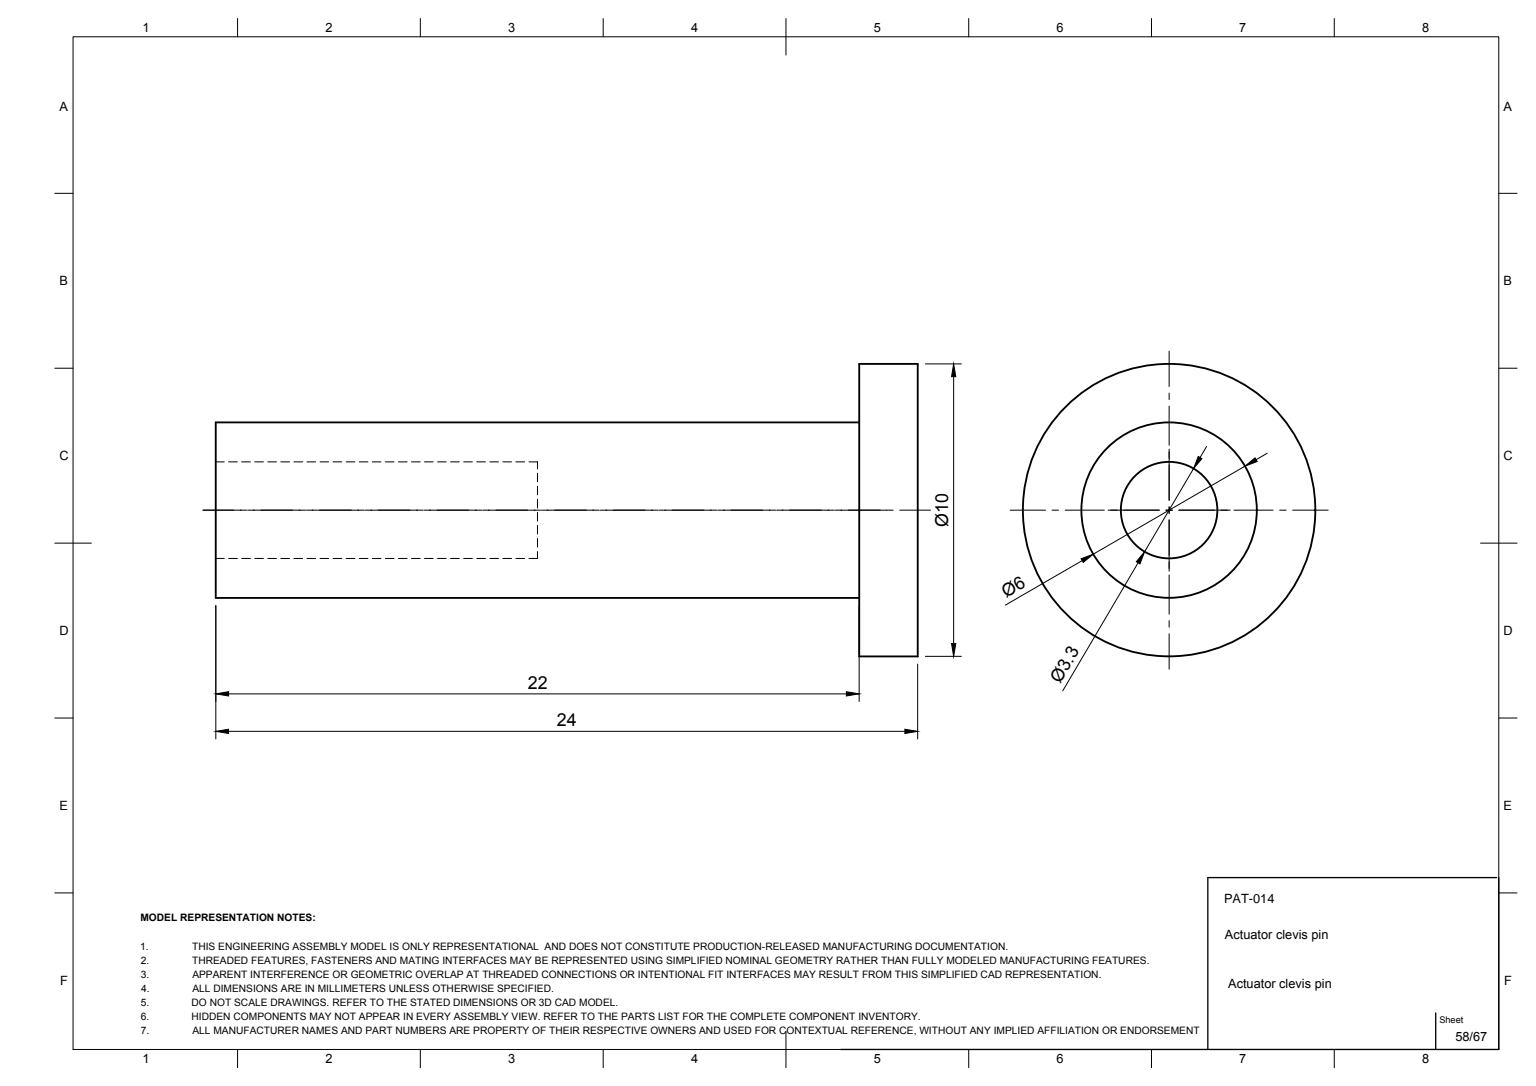
ISO-10303-21;
HEADER;
/* Generated by software containing ST-Developer
 * from STEP Tools, Inc. (www.steptools.com) 
 */

FILE_DESCRIPTION(
/* description */ ('Bin tilter linkage'),
/* implementation_level */ '2;1');

FILE_NAME(
/* name */ 'Actuator clevis pin.step',
/* time_stamp */ '2026-10-28T03:26:24-07:00',
/* author */ (''),
/* organization */ (''),
/* preprocessor_version */ 'ST-DEVELOPER v20.2',
/* originating_system */ 'Autodesk Translation Framework v15.17.0.0',
/* authorisation */ '');

FILE_SCHEMA (('AUTOMOTIVE_DESIGN { 1 0 10303 214 3 1 1 }'));
ENDSEC;

DATA;
#10=MECHANICAL_DESIGN_GEOMETRIC_PRESENTATION_REPRESENTATION('',(#964),#23728);
#744=SHAPE_REPRESENTATION_RELATIONSHIP('SRR','None',#24213,#850);
#850=ADVANCED_BREP_SHAPE_REPRESENTATION('',(#1076),#23713);
#964=STYLED_ITEM('',(#24765),#1076);
#1076=MANIFOLD_SOLID_BREP('Body1',#12496);
#1464=FACE_BOUND('',#3742,.T.);
#1465=FACE_BOUND('',#3747,.T.);
#1840=PLANE('',#15289);
#1841=PLANE('',#15290);
#1842=PLANE('',#15295);
#1843=PLANE('',#15298);
#2585=FACE_OUTER_BOUND('',#3739,.T.);
#2586=FACE_OUTER_BOUND('',#3740,.T.);
#2587=FACE_OUTER_BOUND('',#3741,.T.);
#2588=FACE_OUTER_BOUND('',#3743,.T.);
#2589=FACE_OUTER_BOUND('',#3744,.T.);
#2590=FACE_OUTER_BOUND('',#3745,.T.);
#2591=FACE_OUTER_BOUND('',#3746,.T.);
#3739=EDGE_LOOP('',(#10985,#10986,#10987,#10988));
#3740=EDGE_LOOP('',(#10989));
#3741=EDGE_LOOP('',(#10990));
#3742=EDGE_LOOP('',(#10991));
#3743=EDGE_LOOP('',(#10992,#10993,#10994,#10995));
#3744=EDGE_LOOP('',(#10996));
#3745=EDGE_LOOP('',(#10997,#10998,#10999,#11000));
#3746=EDGE_LOOP('',(#11001));
#3747=EDGE_LOOP('',(#11002));
#4450=LINE('',#23144,#5125);
#4451=LINE('',#23154,#5126);
#4452=LINE('',#23160,#5127);
#5125=VECTOR('',#19299,0.165);
#5126=VECTOR('',#19312,0.5);
#5127=VECTOR('',#19321,0.3);
#5890=CIRCLE('',#15287,0.165);
#5891=CIRCLE('',#15288,0.165);
#5892=CIRCLE('',#15291,0.5);
#5893=CIRCLE('',#15292,0.3);
#5894=CIRCLE('',#15294,0.5);
#5895=CIRCLE('',#15297,0.3);
#6833=VERTEX_POINT('',#23141);
#6834=VERTEX_POINT('',#23143);
#6835=VERTEX_POINT('',#23148);
#6836=VERTEX_POINT('',#23150);
#6837=VERTEX_POINT('',#23153);
#6838=VERTEX_POINT('',#23158);
#8232=EDGE_CURVE('',#6833,#6833,#5890,.T.);
#8233=EDGE_CURVE('',#6833,#6834,#4450,.T.);
#8234=EDGE_CURVE('',#6834,#6834,#5891,.T.);
#8235=EDGE_CURVE('',#6835,#6835,#5892,.T.);
#8236=EDGE_CURVE('',#6836,#6836,#5893,.T.);
#8237=EDGE_CURVE('',#6835,#6837,#4451,.T.);
#8238=EDGE_CURVE('',#6837,#6837,#5894,.T.);
#8239=EDGE_CURVE('',#6838,#6838,#5895,.T.);
#8240=EDGE_CURVE('',#6838,#6836,#4452,.T.);
#10985=ORIENTED_EDGE('',*,*,#8232,.F.);
#10986=ORIENTED_EDGE('',*,*,#8233,.T.);
#10987=ORIENTED_EDGE('',*,*,#8234,.F.);
#10988=ORIENTED_EDGE('',*,*,#8233,.F.);
#10989=ORIENTED_EDGE('',*,*,#8232,.T.);
#10990=ORIENTED_EDGE('',*,*,#8235,.T.);
#10991=ORIENTED_EDGE('',*,*,#8236,.F.);
#10992=ORIENTED_EDGE('',*,*,#8235,.F.);
#10993=ORIENTED_EDGE('',*,*,#8237,.T.);
#10994=ORIENTED_EDGE('',*,*,#8238,.T.);
#10995=ORIENTED_EDGE('',*,*,#8237,.F.);
#10996=ORIENTED_EDGE('',*,*,#8238,.F.);
#10997=ORIENTED_EDGE('',*,*,#8239,.F.);
#10998=ORIENTED_EDGE('',*,*,#8240,.T.);
#10999=ORIENTED_EDGE('',*,*,#8236,.T.);
#11000=ORIENTED_EDGE('',*,*,#8240,.F.);
#11001=ORIENTED_EDGE('',*,*,#8239,.T.);
#11002=ORIENTED_EDGE('',*,*,#8234,.T.);
#11586=CYLINDRICAL_SURFACE('',#15286,0.165);
#11587=CYLINDRICAL_SURFACE('',#15293,0.5);
#11588=CYLINDRICAL_SURFACE('',#15296,0.3);
#12310=ADVANCED_FACE('',(#2585),#11586,.F.);
#12311=ADVANCED_FACE('',(#2586),#1840,.T.);
#12312=ADVANCED_FACE('',(#2587,#1464),#1841,.T.);
#12313=ADVANCED_FACE('',(#2588),#11587,.T.);
#12314=ADVANCED_FACE('',(#2589),#1842,.F.);
#12315=ADVANCED_FACE('',(#2590),#11588,.T.);
#12316=ADVANCED_FACE('',(#2591,#1465),#1843,.T.);
#12496=CLOSED_SHELL('',(#12310,#12311,#12312,#12313,#12314,#12315,#12316));
#15285=AXIS2_PLACEMENT_3D('',#23139,#19293,#19294);
#15286=AXIS2_PLACEMENT_3D('',#23140,#19295,#19296);
#15287=AXIS2_PLACEMENT_3D('',#23142,#19297,#19298);
#15288=AXIS2_PLACEMENT_3D('',#23145,#19300,#19301);
#15289=AXIS2_PLACEMENT_3D('',#23146,#19302,#19303);
#15290=AXIS2_PLACEMENT_3D('',#23147,#19304,#19305);
#15291=AXIS2_PLACEMENT_3D('',#23149,#19306,#19307);
#15292=AXIS2_PLACEMENT_3D('',#23151,#19308,#19309);
#15293=AXIS2_PLACEMENT_3D('',#23152,#19310,#19311);
#15294=AXIS2_PLACEMENT_3D('',#23155,#19313,#19314);
#15295=AXIS2_PLACEMENT_3D('',#23156,#19315,#19316);
#15296=AXIS2_PLACEMENT_3D('',#23157,#19317,#19318);
#15297=AXIS2_PLACEMENT_3D('',#23159,#19319,#19320);
#15298=AXIS2_PLACEMENT_3D('',#23161,#19322,#19323);
#19293=DIRECTION('axis',(0.,0.,1.));
#19294=DIRECTION('refdir',(1.,0.,0.));
#19295=DIRECTION('center_axis',(0.,1.,0.));
#19296=DIRECTION('ref_axis',(1.,0.,0.));
#19297=DIRECTION('center_axis',(0.,1.,0.));
#19298=DIRECTION('ref_axis',(1.,0.,0.));
#19299=DIRECTION('',(0.,1.,0.));
#19300=DIRECTION('center_axis',(0.,-1.,0.));
#19301=DIRECTION('ref_axis',(1.,0.,0.));
#19302=DIRECTION('center_axis',(0.,1.,0.));
#19303=DIRECTION('ref_axis',(1.,0.,0.));
#19304=DIRECTION('center_axis',(0.,1.,0.));
#19305=DIRECTION('ref_axis',(1.,0.,0.));
#19306=DIRECTION('center_axis',(0.,1.,0.));
#19307=DIRECTION('ref_axis',(1.,0.,0.));
#19308=DIRECTION('center_axis',(0.,1.,0.));
#19309=DIRECTION('ref_axis',(1.,0.,0.));
#19310=DIRECTION('center_axis',(0.,1.,0.));
#19311=DIRECTION('ref_axis',(1.,0.,0.));
#19312=DIRECTION('',(0.,-1.,0.));
#19313=DIRECTION('center_axis',(0.,1.,0.));
#19314=DIRECTION('ref_axis',(1.,0.,0.));
#19315=DIRECTION('center_axis',(0.,1.,0.));
#19316=DIRECTION('ref_axis',(1.,0.,0.));
#19317=DIRECTION('center_axis',(0.,1.,0.));
#19318=DIRECTION('ref_axis',(1.,0.,0.));
#19319=DIRECTION('center_axis',(0.,1.,0.));
#19320=DIRECTION('ref_axis',(1.,0.,0.));
#19321=DIRECTION('',(0.,-1.,0.));
#19322=DIRECTION('center_axis',(0.,1.,0.));
#19323=DIRECTION('ref_axis',(1.,0.,0.));
#23139=CARTESIAN_POINT('',(0.,0.,0.));
#23140=CARTESIAN_POINT('Origin',(-4.,-4.1,11.));
#23141=CARTESIAN_POINT('',(-4.165,-4.1,11.));
#23142=CARTESIAN_POINT('Origin',(-4.,-4.1,11.));
#23143=CARTESIAN_POINT('',(-4.165,-3.,11.));
#23144=CARTESIAN_POINT('',(-4.165,-4.1,11.));
#23145=CARTESIAN_POINT('Origin',(-4.,-3.,11.));
#23146=CARTESIAN_POINT('Origin',(-4.,-4.1,11.));
#23147=CARTESIAN_POINT('Origin',(-4.,-5.2,11.));
#23148=CARTESIAN_POINT('',(-4.5,-5.2,11.));
#23149=CARTESIAN_POINT('Origin',(-4.,-5.2,11.));
#23150=CARTESIAN_POINT('',(-4.3,-5.2,11.));
#23151=CARTESIAN_POINT('Origin',(-4.,-5.2,11.));
#23152=CARTESIAN_POINT('Origin',(-4.,-5.4,11.));
#23153=CARTESIAN_POINT('',(-4.5,-5.4,11.));
#23154=CARTESIAN_POINT('',(-4.5,-5.4,11.));
#23155=CARTESIAN_POINT('Origin',(-4.,-5.4,11.));
#23156=CARTESIAN_POINT('Origin',(-4.,-5.4,11.));
#23157=CARTESIAN_POINT('Origin',(-4.,-5.2,11.));
#23158=CARTESIAN_POINT('',(-4.3,-3.,11.));
#23159=CARTESIAN_POINT('Origin',(-4.,-3.,11.));
#23160=CARTESIAN_POINT('',(-4.3,-5.2,11.));
#23161=CARTESIAN_POINT('Origin',(-4.,-3.,11.));
#23596=UNCERTAINTY_MEASURE_WITH_UNIT(LENGTH_MEASURE(0.001),#23729,
'DISTANCE_ACCURACY_VALUE',
'Maximum model space distance between geometric entities at asserted c
onnectivities');
#23611=UNCERTAINTY_MEASURE_WITH_UNIT(LENGTH_MEASURE(0.001),#23729,
'DISTANCE_ACCURACY_VALUE',
'Maximum model space distance between geometric entities at asserted c
onnectivities');
#23713=(
GEOMETRIC_REPRESENTATION_CONTEXT(3)
GLOBAL_UNCERTAINTY_ASSIGNED_CONTEXT((#23596))
GLOBAL_UNIT_ASSIGNED_CONTEXT((#23729,#23731,#23732))
REPRESENTATION_CONTEXT('','3D')
);
#23728=(
GEOMETRIC_REPRESENTATION_CONTEXT(3)
GLOBAL_UNCERTAINTY_ASSIGNED_CONTEXT((#23611))
GLOBAL_UNIT_ASSIGNED_CONTEXT((#23729,#23731,#23732))
REPRESENTATION_CONTEXT('','3D')
);
#23729=(
LENGTH_UNIT()
NAMED_UNIT(*)
SI_UNIT(.CENTI.,.METRE.)
);
#23731=(
NAMED_UNIT(*)
PLANE_ANGLE_UNIT()
SI_UNIT($,.RADIAN.)
);
#23732=(
NAMED_UNIT(*)
SI_UNIT($,.STERADIAN.)
SOLID_ANGLE_UNIT()
);
#23834=SHAPE_DEFINITION_REPRESENTATION(#24072,#24213);
#24072=PRODUCT_DEFINITION_SHAPE('',$,#24330);
#24213=SHAPE_REPRESENTATION('',(#15285),#23713);
#24228=PRODUCT_DEFINITION_CONTEXT('part definition',#24578,'design');
#24330=PRODUCT_DEFINITION('Actuator clevis pin','Actuator clevis pin',#24446,
#24228);
#24446=PRODUCT_DEFINITION_FORMATION('',$,#24681);
#24578=APPLICATION_CONTEXT(
'Core Data for Automotive Mechanical Design Process');
#24579=PRODUCT_CONTEXT('part definition',#24578,'mechanical');
#24681=PRODUCT('Actuator clevis pin','Actuator clevis pin',
'Actuator clevis pin',(#24579));
#24759=COLOUR_RGB('Grey',0.48,0.52,0.57);
#24760=FILL_AREA_STYLE_COLOUR('',#24759);
#24761=FILL_AREA_STYLE('',(#24760));
#24762=SURFACE_STYLE_FILL_AREA(#24761);
#24763=SURFACE_SIDE_STYLE('',(#24762));
#24764=SURFACE_STYLE_USAGE(.BOTH.,#24763);
#24765=PRESENTATION_STYLE_ASSIGNMENT((#24764));
ENDSEC;
END-ISO-10303-21;
